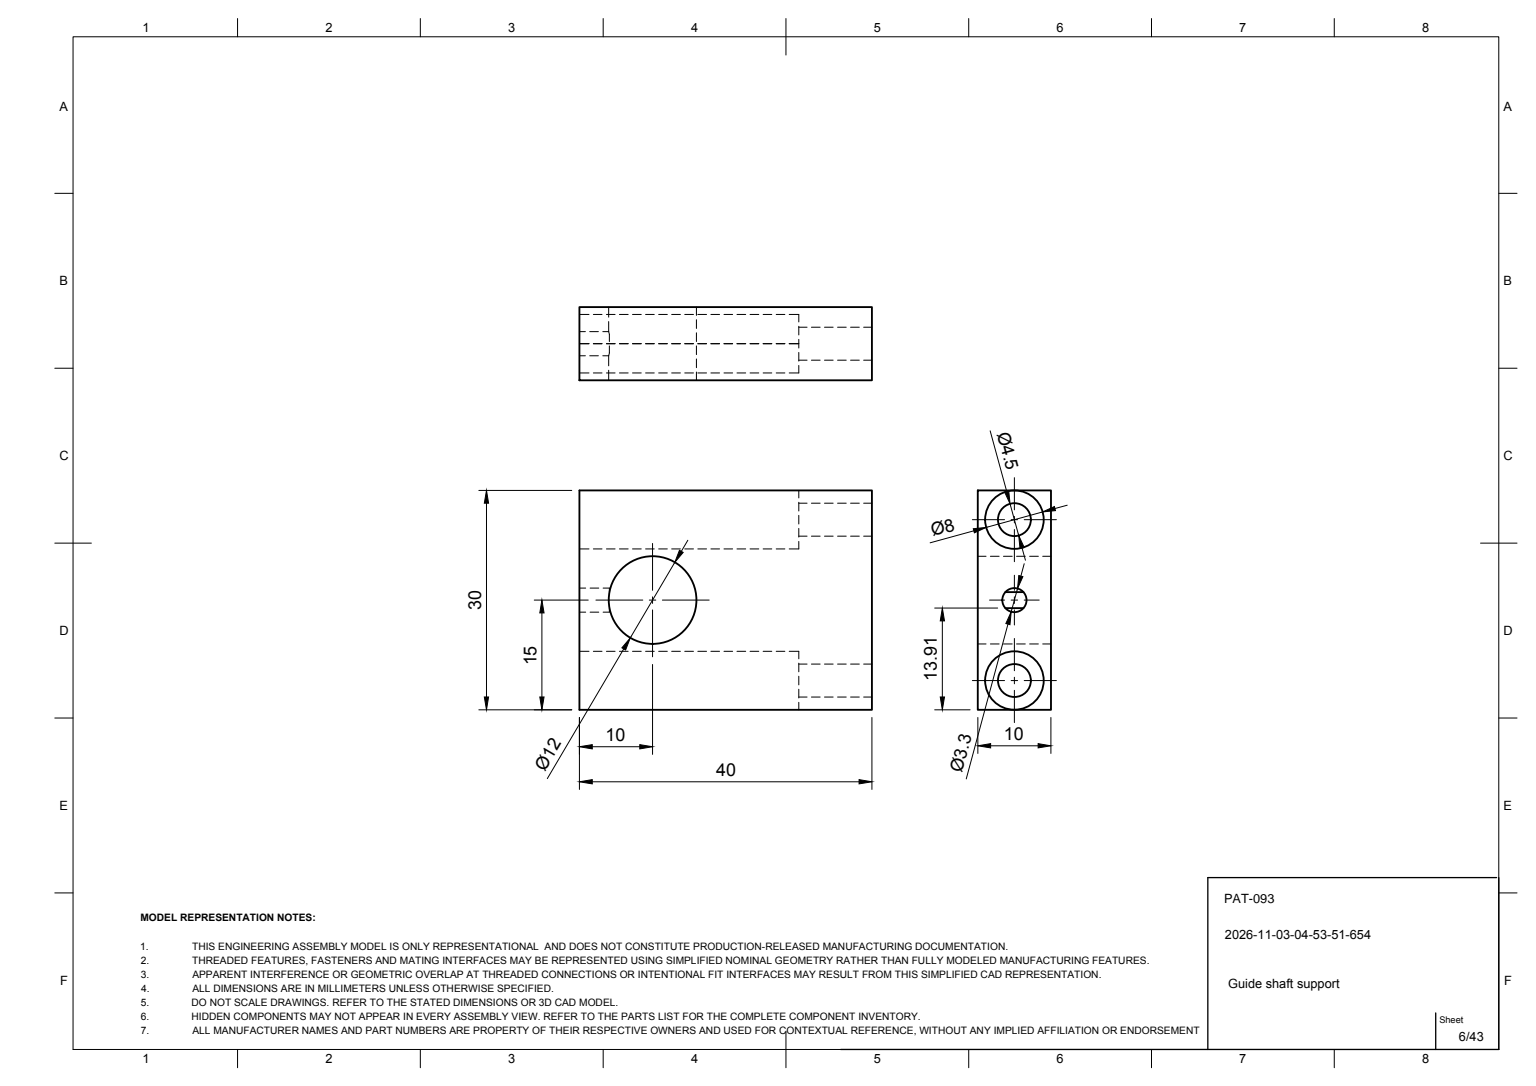
ISO-10303-21;
HEADER;
/* Generated by software containing ST-Developer
 * from STEP Tools, Inc. (www.steptools.com) 
 */

FILE_DESCRIPTION(
/* description */ ('Self-centering screw clamp'),
/* implementation_level */ '2;1');

FILE_NAME(
/* name */ 'Guide shaft support.step',
/* time_stamp */ '2026-10-28T03:25:31-07:00',
/* author */ (''),
/* organization */ (''),
/* preprocessor_version */ 'ST-DEVELOPER v20.2',
/* originating_system */ 'Autodesk Translation Framework v15.17.0.0',
/* authorisation */ '');

FILE_SCHEMA (('AUTOMOTIVE_DESIGN { 1 0 10303 214 3 1 1 }'));
ENDSEC;

DATA;
#10=MECHANICAL_DESIGN_GEOMETRIC_PRESENTATION_REPRESENTATION('',(#627),#16799);
#498=B_SPLINE_CURVE_WITH_KNOTS('',3,(#13857,#13858,#13859,#13860,#13861,
#13862),.UNSPECIFIED.,.F.,.F.,(4,2,4),(0.63543032495593,0.687528937234027,
0.750024497760672),.UNSPECIFIED.);
#499=B_SPLINE_CURVE_WITH_KNOTS('',3,(#13866,#13867,#13868,#13869,#13870,
#13871),.UNSPECIFIED.,.F.,.F.,(4,2,4),(0.250008165920224,0.312503726446869,
0.364602338724965),.UNSPECIFIED.);
#500=B_SPLINE_CURVE_WITH_KNOTS('',3,(#13872,#13873,#13874,#13875,#13876,
#13877),.UNSPECIFIED.,.F.,.F.,(4,2,4),(0.135413993115483,0.187512605393579,
0.250008165920224),.UNSPECIFIED.);
#501=B_SPLINE_CURVE_WITH_KNOTS('',3,(#13878,#13879,#13880,#13881,#13882,
#13883),.UNSPECIFIED.,.F.,.F.,(4,2,4),(0.750024497760672,0.812520058287317,
0.864618670565412),.UNSPECIFIED.);
#545=SHAPE_REPRESENTATION_RELATIONSHIP('SRR','None',#17018,#586);
#586=ADVANCED_BREP_SHAPE_REPRESENTATION('',(#675),#16756);
#627=STYLED_ITEM('',(#17326),#675);
#675=MANIFOLD_SOLID_BREP('Body1',#9078);
#742=FACE_BOUND('',#1838,.T.);
#743=FACE_BOUND('',#1841,.T.);
#744=FACE_BOUND('',#1843,.T.);
#745=FACE_BOUND('',#1849,.T.);
#746=FACE_BOUND('',#1852,.T.);
#747=FACE_BOUND('',#1854,.T.);
#748=FACE_BOUND('',#1855,.T.);
#1032=PLANE('',#9643);
#1033=PLANE('',#9648);
#1034=PLANE('',#9652);
#1035=PLANE('',#9657);
#1036=PLANE('',#9659);
#1037=PLANE('',#9667);
#1038=PLANE('',#9668);
#1039=PLANE('',#9669);
#1040=PLANE('',#9670);
#1041=PLANE('',#9671);
#1303=FACE_OUTER_BOUND('',#1831,.T.);
#1304=FACE_OUTER_BOUND('',#1832,.T.);
#1305=FACE_OUTER_BOUND('',#1833,.T.);
#1306=FACE_OUTER_BOUND('',#1834,.T.);
#1307=FACE_OUTER_BOUND('',#1835,.T.);
#1308=FACE_OUTER_BOUND('',#1836,.T.);
#1309=FACE_OUTER_BOUND('',#1837,.T.);
#1310=FACE_OUTER_BOUND('',#1839,.T.);
#1311=FACE_OUTER_BOUND('',#1840,.T.);
#1312=FACE_OUTER_BOUND('',#1842,.T.);
#1313=FACE_OUTER_BOUND('',#1844,.T.);
#1314=FACE_OUTER_BOUND('',#1845,.T.);
#1315=FACE_OUTER_BOUND('',#1846,.T.);
#1316=FACE_OUTER_BOUND('',#1847,.T.);
#1317=FACE_OUTER_BOUND('',#1848,.T.);
#1318=FACE_OUTER_BOUND('',#1850,.T.);
#1319=FACE_OUTER_BOUND('',#1851,.T.);
#1320=FACE_OUTER_BOUND('',#1853,.T.);
#1831=EDGE_LOOP('',(#6247,#6248,#6249,#6250));
#1832=EDGE_LOOP('',(#6251,#6252,#6253,#6254));
#1833=EDGE_LOOP('',(#6255,#6256));
#1834=EDGE_LOOP('',(#6257,#6258,#6259,#6260,#6261,#6262,#6263,#6264,#6265));
#1835=EDGE_LOOP('',(#6266,#6267));
#1836=EDGE_LOOP('',(#6268,#6269,#6270,#6271));
#1837=EDGE_LOOP('',(#6272,#6273));
#1838=EDGE_LOOP('',(#6274));
#1839=EDGE_LOOP('',(#6275,#6276,#6277,#6278));
#1840=EDGE_LOOP('',(#6279,#6280));
#1841=EDGE_LOOP('',(#6281));
#1842=EDGE_LOOP('',(#6282,#6283,#6284,#6285,#6286,#6287,#6288,#6289,#6290,
#6291));
#1843=EDGE_LOOP('',(#6292));
#1844=EDGE_LOOP('',(#6293,#6294,#6295,#6296));
#1845=EDGE_LOOP('',(#6297,#6298,#6299,#6300));
#1846=EDGE_LOOP('',(#6301,#6302,#6303,#6304,#6305,#6306,#6307,#6308,#6309,
#6310,#6311,#6312));
#1847=EDGE_LOOP('',(#6313,#6314,#6315,#6316,#6317,#6318,#6319));
#1848=EDGE_LOOP('',(#6320,#6321,#6322,#6323));
#1849=EDGE_LOOP('',(#6324));
#1850=EDGE_LOOP('',(#6325,#6326,#6327,#6328,#6329,#6330,#6331));
#1851=EDGE_LOOP('',(#6332,#6333,#6334,#6335));
#1852=EDGE_LOOP('',(#6336));
#1853=EDGE_LOOP('',(#6337,#6338,#6339,#6340));
#1854=EDGE_LOOP('',(#6341));
#1855=EDGE_LOOP('',(#6342));
#2625=LINE('',#13834,#3198);
#2626=LINE('',#13838,#3199);
#2627=LINE('',#13843,#3200);
#2628=LINE('',#13847,#3201);
#2629=LINE('',#13852,#3202);
#2630=LINE('',#13885,#3203);
#2631=LINE('',#13888,#3204);
#2632=LINE('',#13891,#3205);
#2633=LINE('',#13898,#3206);
#2634=LINE('',#13906,#3207);
#2635=LINE('',#13907,#3208);
#2636=LINE('',#13909,#3209);
#2637=LINE('',#13911,#3210);
#2638=LINE('',#13912,#3211);
#2639=LINE('',#13913,#3212);
#2640=LINE('',#13917,#3213);
#2641=LINE('',#13921,#3214);
#2642=LINE('',#13925,#3215);
#2643=LINE('',#13927,#3216);
#2644=LINE('',#13932,#3217);
#2645=LINE('',#13933,#3218);
#2646=LINE('',#13934,#3219);
#2647=LINE('',#13937,#3220);
#2648=LINE('',#13938,#3221);
#2649=LINE('',#13941,#3222);
#2650=LINE('',#13942,#3223);
#2651=LINE('',#13944,#3224);
#3198=VECTOR('',#10922,0.4);
#3199=VECTOR('',#10925,1.);
#3200=VECTOR('',#10930,0.4);
#3201=VECTOR('',#10933,1.);
#3202=VECTOR('',#10938,1.);
#3203=VECTOR('',#10945,0.164999999999999);
#3204=VECTOR('',#10950,1.);
#3205=VECTOR('',#10955,1.);
#3206=VECTOR('',#10966,1.);
#3207=VECTOR('',#10975,1.);
#3208=VECTOR('',#10976,1.);
#3209=VECTOR('',#10977,1.);
#3210=VECTOR('',#10978,1.);
#3211=VECTOR('',#10979,1.);
#3212=VECTOR('',#10980,1.);
#3213=VECTOR('',#10985,0.225);
#3214=VECTOR('',#10990,0.225);
#3215=VECTOR('',#10995,0.6);
#3216=VECTOR('',#10996,0.6);
#3217=VECTOR('',#11001,1.);
#3218=VECTOR('',#11002,1.);
#3219=VECTOR('',#11003,1.);
#3220=VECTOR('',#11006,1.);
#3221=VECTOR('',#11007,1.);
#3222=VECTOR('',#11010,1.);
#3223=VECTOR('',#11011,1.);
#3224=VECTOR('',#11014,1.);
#3747=CIRCLE('',#9638,0.4);
#3748=CIRCLE('',#9639,0.4);
#3749=CIRCLE('',#9641,0.4);
#3750=CIRCLE('',#9642,0.4);
#3751=CIRCLE('',#9644,0.164999999999999);
#3752=CIRCLE('',#9646,0.164999999999999);
#3753=CIRCLE('',#9647,0.164999999999999);
#3754=CIRCLE('',#9650,0.4);
#3755=CIRCLE('',#9651,0.4);
#3756=CIRCLE('',#9653,0.225);
#3757=CIRCLE('',#9655,0.4);
#3758=CIRCLE('',#9656,0.4);
#3759=CIRCLE('',#9658,0.225);
#3760=CIRCLE('',#9661,0.225);
#3761=CIRCLE('',#9663,0.225);
#3762=CIRCLE('',#9665,0.6);
#3763=CIRCLE('',#9666,0.6);
#4281=VERTEX_POINT('',#13832);
#4282=VERTEX_POINT('',#13833);
#4283=VERTEX_POINT('',#13835);
#4284=VERTEX_POINT('',#13837);
#4285=VERTEX_POINT('',#13841);
#4286=VERTEX_POINT('',#13842);
#4287=VERTEX_POINT('',#13844);
#4288=VERTEX_POINT('',#13846);
#4289=VERTEX_POINT('',#13850);
#4290=VERTEX_POINT('',#13851);
#4291=VERTEX_POINT('',#13855);
#4292=VERTEX_POINT('',#13856);
#4293=VERTEX_POINT('',#13863);
#4294=VERTEX_POINT('',#13865);
#4295=VERTEX_POINT('',#13884);
#4296=VERTEX_POINT('',#13894);
#4297=VERTEX_POINT('',#13901);
#4298=VERTEX_POINT('',#13904);
#4299=VERTEX_POINT('',#13905);
#4300=VERTEX_POINT('',#13908);
#4301=VERTEX_POINT('',#13910);
#4302=VERTEX_POINT('',#13915);
#4303=VERTEX_POINT('',#13919);
#4304=VERTEX_POINT('',#13923);
#4305=VERTEX_POINT('',#13926);
#4306=VERTEX_POINT('',#13930);
#4307=VERTEX_POINT('',#13931);
#4308=VERTEX_POINT('',#13936);
#4309=VERTEX_POINT('',#13940);
#5048=EDGE_CURVE('',#4281,#4282,#2625,.T.);
#5049=EDGE_CURVE('',#4283,#4281,#3747,.T.);
#5050=EDGE_CURVE('',#4283,#4284,#2626,.T.);
#5051=EDGE_CURVE('',#4282,#4284,#3748,.T.);
#5052=EDGE_CURVE('',#4285,#4286,#2627,.T.);
#5053=EDGE_CURVE('',#4287,#4285,#3749,.T.);
#5054=EDGE_CURVE('',#4287,#4288,#2628,.T.);
#5055=EDGE_CURVE('',#4286,#4288,#3750,.T.);
#5056=EDGE_CURVE('',#4289,#4290,#2629,.T.);
#5057=EDGE_CURVE('',#4289,#4290,#3751,.T.);
#5058=EDGE_CURVE('',#4291,#4292,#498,.T.);
#5059=EDGE_CURVE('',#4293,#4291,#3752,.T.);
#5060=EDGE_CURVE('',#4294,#4293,#499,.T.);
#5061=EDGE_CURVE('',#4290,#4294,#500,.T.);
#5062=EDGE_CURVE('',#4292,#4289,#501,.T.);
#5063=EDGE_CURVE('',#4292,#4295,#2630,.T.);
#5064=EDGE_CURVE('',#4295,#4295,#3753,.T.);
#5065=EDGE_CURVE('',#4293,#4291,#2631,.T.);
#5066=EDGE_CURVE('',#4288,#4286,#3754,.T.);
#5067=EDGE_CURVE('',#4287,#4288,#2632,.T.);
#5068=EDGE_CURVE('',#4285,#4287,#3755,.T.);
#5069=EDGE_CURVE('',#4296,#4296,#3756,.T.);
#5070=EDGE_CURVE('',#4284,#4282,#3757,.T.);
#5071=EDGE_CURVE('',#4283,#4284,#2633,.T.);
#5072=EDGE_CURVE('',#4281,#4283,#3758,.T.);
#5073=EDGE_CURVE('',#4297,#4297,#3759,.T.);
#5074=EDGE_CURVE('',#4298,#4299,#2634,.T.);
#5075=EDGE_CURVE('',#4299,#4288,#2635,.T.);
#5076=EDGE_CURVE('',#4288,#4300,#2636,.T.);
#5077=EDGE_CURVE('',#4300,#4301,#2637,.T.);
#5078=EDGE_CURVE('',#4301,#4284,#2638,.T.);
#5079=EDGE_CURVE('',#4284,#4298,#2639,.T.);
#5080=EDGE_CURVE('',#4302,#4302,#3760,.T.);
#5081=EDGE_CURVE('',#4302,#4296,#2640,.T.);
#5082=EDGE_CURVE('',#4303,#4303,#3761,.T.);
#5083=EDGE_CURVE('',#4303,#4297,#2641,.T.);
#5084=EDGE_CURVE('',#4304,#4304,#3762,.T.);
#5085=EDGE_CURVE('',#4304,#4292,#2642,.T.);
#5086=EDGE_CURVE('',#4294,#4305,#2643,.T.);
#5087=EDGE_CURVE('',#4305,#4305,#3763,.T.);
#5088=EDGE_CURVE('',#4306,#4307,#2644,.T.);
#5089=EDGE_CURVE('',#4307,#4298,#2645,.T.);
#5090=EDGE_CURVE('',#4306,#4301,#2646,.T.);
#5091=EDGE_CURVE('',#4308,#4306,#2647,.T.);
#5092=EDGE_CURVE('',#4308,#4300,#2648,.T.);
#5093=EDGE_CURVE('',#4309,#4308,#2649,.T.);
#5094=EDGE_CURVE('',#4309,#4299,#2650,.T.);
#5095=EDGE_CURVE('',#4307,#4309,#2651,.T.);
#6247=ORIENTED_EDGE('',*,*,#5048,.F.);
#6248=ORIENTED_EDGE('',*,*,#5049,.F.);
#6249=ORIENTED_EDGE('',*,*,#5050,.T.);
#6250=ORIENTED_EDGE('',*,*,#5051,.F.);
#6251=ORIENTED_EDGE('',*,*,#5052,.F.);
#6252=ORIENTED_EDGE('',*,*,#5053,.F.);
#6253=ORIENTED_EDGE('',*,*,#5054,.T.);
#6254=ORIENTED_EDGE('',*,*,#5055,.F.);
#6255=ORIENTED_EDGE('',*,*,#5056,.F.);
#6256=ORIENTED_EDGE('',*,*,#5057,.T.);
#6257=ORIENTED_EDGE('',*,*,#5058,.F.);
#6258=ORIENTED_EDGE('',*,*,#5059,.F.);
#6259=ORIENTED_EDGE('',*,*,#5060,.F.);
#6260=ORIENTED_EDGE('',*,*,#5061,.F.);
#6261=ORIENTED_EDGE('',*,*,#5057,.F.);
#6262=ORIENTED_EDGE('',*,*,#5062,.F.);
#6263=ORIENTED_EDGE('',*,*,#5063,.T.);
#6264=ORIENTED_EDGE('',*,*,#5064,.F.);
#6265=ORIENTED_EDGE('',*,*,#5063,.F.);
#6266=ORIENTED_EDGE('',*,*,#5065,.F.);
#6267=ORIENTED_EDGE('',*,*,#5059,.T.);
#6268=ORIENTED_EDGE('',*,*,#5052,.T.);
#6269=ORIENTED_EDGE('',*,*,#5066,.F.);
#6270=ORIENTED_EDGE('',*,*,#5067,.F.);
#6271=ORIENTED_EDGE('',*,*,#5068,.F.);
#6272=ORIENTED_EDGE('',*,*,#5053,.T.);
#6273=ORIENTED_EDGE('',*,*,#5068,.T.);
#6274=ORIENTED_EDGE('',*,*,#5069,.F.);
#6275=ORIENTED_EDGE('',*,*,#5048,.T.);
#6276=ORIENTED_EDGE('',*,*,#5070,.F.);
#6277=ORIENTED_EDGE('',*,*,#5071,.F.);
#6278=ORIENTED_EDGE('',*,*,#5072,.F.);
#6279=ORIENTED_EDGE('',*,*,#5049,.T.);
#6280=ORIENTED_EDGE('',*,*,#5072,.T.);
#6281=ORIENTED_EDGE('',*,*,#5073,.F.);
#6282=ORIENTED_EDGE('',*,*,#5074,.T.);
#6283=ORIENTED_EDGE('',*,*,#5075,.T.);
#6284=ORIENTED_EDGE('',*,*,#5066,.T.);
#6285=ORIENTED_EDGE('',*,*,#5055,.T.);
#6286=ORIENTED_EDGE('',*,*,#5076,.T.);
#6287=ORIENTED_EDGE('',*,*,#5077,.T.);
#6288=ORIENTED_EDGE('',*,*,#5078,.T.);
#6289=ORIENTED_EDGE('',*,*,#5070,.T.);
#6290=ORIENTED_EDGE('',*,*,#5051,.T.);
#6291=ORIENTED_EDGE('',*,*,#5079,.T.);
#6292=ORIENTED_EDGE('',*,*,#5064,.T.);
#6293=ORIENTED_EDGE('',*,*,#5080,.F.);
#6294=ORIENTED_EDGE('',*,*,#5081,.T.);
#6295=ORIENTED_EDGE('',*,*,#5069,.T.);
#6296=ORIENTED_EDGE('',*,*,#5081,.F.);
#6297=ORIENTED_EDGE('',*,*,#5082,.F.);
#6298=ORIENTED_EDGE('',*,*,#5083,.T.);
#6299=ORIENTED_EDGE('',*,*,#5073,.T.);
#6300=ORIENTED_EDGE('',*,*,#5083,.F.);
#6301=ORIENTED_EDGE('',*,*,#5084,.F.);
#6302=ORIENTED_EDGE('',*,*,#5085,.T.);
#6303=ORIENTED_EDGE('',*,*,#5062,.T.);
#6304=ORIENTED_EDGE('',*,*,#5056,.T.);
#6305=ORIENTED_EDGE('',*,*,#5061,.T.);
#6306=ORIENTED_EDGE('',*,*,#5086,.T.);
#6307=ORIENTED_EDGE('',*,*,#5087,.F.);
#6308=ORIENTED_EDGE('',*,*,#5086,.F.);
#6309=ORIENTED_EDGE('',*,*,#5060,.T.);
#6310=ORIENTED_EDGE('',*,*,#5065,.T.);
#6311=ORIENTED_EDGE('',*,*,#5058,.T.);
#6312=ORIENTED_EDGE('',*,*,#5085,.F.);
#6313=ORIENTED_EDGE('',*,*,#5088,.T.);
#6314=ORIENTED_EDGE('',*,*,#5089,.T.);
#6315=ORIENTED_EDGE('',*,*,#5079,.F.);
#6316=ORIENTED_EDGE('',*,*,#5050,.F.);
#6317=ORIENTED_EDGE('',*,*,#5071,.T.);
#6318=ORIENTED_EDGE('',*,*,#5078,.F.);
#6319=ORIENTED_EDGE('',*,*,#5090,.F.);
#6320=ORIENTED_EDGE('',*,*,#5091,.T.);
#6321=ORIENTED_EDGE('',*,*,#5090,.T.);
#6322=ORIENTED_EDGE('',*,*,#5077,.F.);
#6323=ORIENTED_EDGE('',*,*,#5092,.F.);
#6324=ORIENTED_EDGE('',*,*,#5087,.T.);
#6325=ORIENTED_EDGE('',*,*,#5093,.T.);
#6326=ORIENTED_EDGE('',*,*,#5092,.T.);
#6327=ORIENTED_EDGE('',*,*,#5076,.F.);
#6328=ORIENTED_EDGE('',*,*,#5054,.F.);
#6329=ORIENTED_EDGE('',*,*,#5067,.T.);
#6330=ORIENTED_EDGE('',*,*,#5075,.F.);
#6331=ORIENTED_EDGE('',*,*,#5094,.F.);
#6332=ORIENTED_EDGE('',*,*,#5095,.T.);
#6333=ORIENTED_EDGE('',*,*,#5094,.T.);
#6334=ORIENTED_EDGE('',*,*,#5074,.F.);
#6335=ORIENTED_EDGE('',*,*,#5089,.F.);
#6336=ORIENTED_EDGE('',*,*,#5084,.T.);
#6337=ORIENTED_EDGE('',*,*,#5095,.F.);
#6338=ORIENTED_EDGE('',*,*,#5088,.F.);
#6339=ORIENTED_EDGE('',*,*,#5091,.F.);
#6340=ORIENTED_EDGE('',*,*,#5093,.F.);
#6341=ORIENTED_EDGE('',*,*,#5080,.T.);
#6342=ORIENTED_EDGE('',*,*,#5082,.T.);
#8369=CYLINDRICAL_SURFACE('',#9637,0.4);
#8370=CYLINDRICAL_SURFACE('',#9640,0.4);
#8371=CYLINDRICAL_SURFACE('',#9645,0.164999999999999);
#8372=CYLINDRICAL_SURFACE('',#9649,0.4);
#8373=CYLINDRICAL_SURFACE('',#9654,0.4);
#8374=CYLINDRICAL_SURFACE('',#9660,0.225);
#8375=CYLINDRICAL_SURFACE('',#9662,0.225);
#8376=CYLINDRICAL_SURFACE('',#9664,0.6);
#8601=ADVANCED_FACE('',(#1303),#8369,.F.);
#8602=ADVANCED_FACE('',(#1304),#8370,.F.);
#8603=ADVANCED_FACE('',(#1305),#1032,.T.);
#8604=ADVANCED_FACE('',(#1306),#8371,.F.);
#8605=ADVANCED_FACE('',(#1307),#1033,.T.);
#8606=ADVANCED_FACE('',(#1308),#8372,.F.);
#8607=ADVANCED_FACE('',(#1309,#742),#1034,.T.);
#8608=ADVANCED_FACE('',(#1310),#8373,.F.);
#8609=ADVANCED_FACE('',(#1311,#743),#1035,.T.);
#8610=ADVANCED_FACE('',(#1312,#744),#1036,.T.);
#8611=ADVANCED_FACE('',(#1313),#8374,.F.);
#8612=ADVANCED_FACE('',(#1314),#8375,.F.);
#8613=ADVANCED_FACE('',(#1315),#8376,.F.);
#8614=ADVANCED_FACE('',(#1316),#1037,.T.);
#8615=ADVANCED_FACE('',(#1317,#745),#1038,.T.);
#8616=ADVANCED_FACE('',(#1318),#1039,.T.);
#8617=ADVANCED_FACE('',(#1319,#746),#1040,.T.);
#8618=ADVANCED_FACE('',(#1320,#747,#748),#1041,.F.);
#9078=CLOSED_SHELL('',(#8601,#8602,#8603,#8604,#8605,#8606,#8607,#8608,
#8609,#8610,#8611,#8612,#8613,#8614,#8615,#8616,#8617,#8618));
#9636=AXIS2_PLACEMENT_3D('',#13830,#10918,#10919);
#9637=AXIS2_PLACEMENT_3D('',#13831,#10920,#10921);
#9638=AXIS2_PLACEMENT_3D('',#13836,#10923,#10924);
#9639=AXIS2_PLACEMENT_3D('',#13839,#10926,#10927);
#9640=AXIS2_PLACEMENT_3D('',#13840,#10928,#10929);
#9641=AXIS2_PLACEMENT_3D('',#13845,#10931,#10932);
#9642=AXIS2_PLACEMENT_3D('',#13848,#10934,#10935);
#9643=AXIS2_PLACEMENT_3D('',#13849,#10936,#10937);
#9644=AXIS2_PLACEMENT_3D('',#13853,#10939,#10940);
#9645=AXIS2_PLACEMENT_3D('',#13854,#10941,#10942);
#9646=AXIS2_PLACEMENT_3D('',#13864,#10943,#10944);
#9647=AXIS2_PLACEMENT_3D('',#13886,#10946,#10947);
#9648=AXIS2_PLACEMENT_3D('',#13887,#10948,#10949);
#9649=AXIS2_PLACEMENT_3D('',#13889,#10951,#10952);
#9650=AXIS2_PLACEMENT_3D('',#13890,#10953,#10954);
#9651=AXIS2_PLACEMENT_3D('',#13892,#10956,#10957);
#9652=AXIS2_PLACEMENT_3D('',#13893,#10958,#10959);
#9653=AXIS2_PLACEMENT_3D('',#13895,#10960,#10961);
#9654=AXIS2_PLACEMENT_3D('',#13896,#10962,#10963);
#9655=AXIS2_PLACEMENT_3D('',#13897,#10964,#10965);
#9656=AXIS2_PLACEMENT_3D('',#13899,#10967,#10968);
#9657=AXIS2_PLACEMENT_3D('',#13900,#10969,#10970);
#9658=AXIS2_PLACEMENT_3D('',#13902,#10971,#10972);
#9659=AXIS2_PLACEMENT_3D('',#13903,#10973,#10974);
#9660=AXIS2_PLACEMENT_3D('',#13914,#10981,#10982);
#9661=AXIS2_PLACEMENT_3D('',#13916,#10983,#10984);
#9662=AXIS2_PLACEMENT_3D('',#13918,#10986,#10987);
#9663=AXIS2_PLACEMENT_3D('',#13920,#10988,#10989);
#9664=AXIS2_PLACEMENT_3D('',#13922,#10991,#10992);
#9665=AXIS2_PLACEMENT_3D('',#13924,#10993,#10994);
#9666=AXIS2_PLACEMENT_3D('',#13928,#10997,#10998);
#9667=AXIS2_PLACEMENT_3D('',#13929,#10999,#11000);
#9668=AXIS2_PLACEMENT_3D('',#13935,#11004,#11005);
#9669=AXIS2_PLACEMENT_3D('',#13939,#11008,#11009);
#9670=AXIS2_PLACEMENT_3D('',#13943,#11012,#11013);
#9671=AXIS2_PLACEMENT_3D('',#13945,#11015,#11016);
#10918=DIRECTION('axis',(0.,0.,1.));
#10919=DIRECTION('refdir',(1.,0.,0.));
#10920=DIRECTION('center_axis',(0.,0.,1.));
#10921=DIRECTION('ref_axis',(1.,0.,0.));
#10922=DIRECTION('',(0.,0.,1.));
#10923=DIRECTION('center_axis',(0.,0.,1.));
#10924=DIRECTION('ref_axis',(1.,0.,0.));
#10925=DIRECTION('',(0.,0.,1.));
#10926=DIRECTION('center_axis',(0.,0.,-1.));
#10927=DIRECTION('ref_axis',(1.,0.,0.));
#10928=DIRECTION('center_axis',(0.,0.,1.));
#10929=DIRECTION('ref_axis',(1.,0.,0.));
#10930=DIRECTION('',(0.,0.,1.));
#10931=DIRECTION('center_axis',(0.,0.,1.));
#10932=DIRECTION('ref_axis',(1.,0.,0.));
#10933=DIRECTION('',(0.,0.,1.));
#10934=DIRECTION('center_axis',(0.,0.,-1.));
#10935=DIRECTION('ref_axis',(1.,0.,0.));
#10936=DIRECTION('center_axis',(0.,0.,1.));
#10937=DIRECTION('ref_axis',(1.,0.,0.));
#10938=DIRECTION('',(1.,0.,0.));
#10939=DIRECTION('center_axis',(0.,0.,1.));
#10940=DIRECTION('ref_axis',(1.,0.,0.));
#10941=DIRECTION('center_axis',(0.,0.,1.));
#10942=DIRECTION('ref_axis',(1.,0.,0.));
#10943=DIRECTION('center_axis',(0.,0.,1.));
#10944=DIRECTION('ref_axis',(1.,0.,0.));
#10945=DIRECTION('',(0.,0.,1.));
#10946=DIRECTION('center_axis',(0.,0.,-1.));
#10947=DIRECTION('ref_axis',(1.,0.,0.));
#10948=DIRECTION('center_axis',(0.,0.,1.));
#10949=DIRECTION('ref_axis',(1.,0.,0.));
#10950=DIRECTION('',(-1.,0.,0.));
#10951=DIRECTION('center_axis',(0.,0.,1.));
#10952=DIRECTION('ref_axis',(1.,0.,0.));
#10953=DIRECTION('center_axis',(0.,0.,-1.));
#10954=DIRECTION('ref_axis',(1.,0.,0.));
#10955=DIRECTION('',(0.,0.,1.));
#10956=DIRECTION('center_axis',(0.,0.,1.));
#10957=DIRECTION('ref_axis',(1.,0.,0.));
#10958=DIRECTION('center_axis',(0.,0.,1.));
#10959=DIRECTION('ref_axis',(1.,0.,0.));
#10960=DIRECTION('center_axis',(0.,0.,1.));
#10961=DIRECTION('ref_axis',(1.,0.,0.));
#10962=DIRECTION('center_axis',(0.,0.,1.));
#10963=DIRECTION('ref_axis',(1.,0.,0.));
#10964=DIRECTION('center_axis',(0.,0.,-1.));
#10965=DIRECTION('ref_axis',(1.,0.,0.));
#10966=DIRECTION('',(0.,0.,1.));
#10967=DIRECTION('center_axis',(0.,0.,1.));
#10968=DIRECTION('ref_axis',(1.,0.,0.));
#10969=DIRECTION('center_axis',(0.,0.,1.));
#10970=DIRECTION('ref_axis',(1.,0.,0.));
#10971=DIRECTION('center_axis',(0.,0.,1.));
#10972=DIRECTION('ref_axis',(1.,0.,0.));
#10973=DIRECTION('center_axis',(0.,0.,1.));
#10974=DIRECTION('ref_axis',(1.,0.,0.));
#10975=DIRECTION('',(0.,-1.,0.));
#10976=DIRECTION('',(1.,0.,0.));
#10977=DIRECTION('',(1.,0.,0.));
#10978=DIRECTION('',(0.,1.,0.));
#10979=DIRECTION('',(-1.,0.,0.));
#10980=DIRECTION('',(-1.,0.,0.));
#10981=DIRECTION('center_axis',(0.,0.,1.));
#10982=DIRECTION('ref_axis',(1.,0.,0.));
#10983=DIRECTION('center_axis',(0.,0.,1.));
#10984=DIRECTION('ref_axis',(1.,0.,0.));
#10985=DIRECTION('',(0.,0.,1.));
#10986=DIRECTION('center_axis',(0.,0.,1.));
#10987=DIRECTION('ref_axis',(1.,0.,0.));
#10988=DIRECTION('center_axis',(0.,0.,1.));
#10989=DIRECTION('ref_axis',(1.,0.,0.));
#10990=DIRECTION('',(0.,0.,1.));
#10991=DIRECTION('center_axis',(1.,0.,0.));
#10992=DIRECTION('ref_axis',(0.,0.,-1.));
#10993=DIRECTION('center_axis',(1.,0.,0.));
#10994=DIRECTION('ref_axis',(0.,0.,-1.));
#10995=DIRECTION('',(1.,0.,0.));
#10996=DIRECTION('',(1.,0.,0.));
#10997=DIRECTION('center_axis',(-1.,0.,0.));
#10998=DIRECTION('ref_axis',(0.,0.,-1.));
#10999=DIRECTION('center_axis',(0.,1.,0.));
#11000=DIRECTION('ref_axis',(-1.,0.,0.));
#11001=DIRECTION('',(-1.,0.,0.));
#11002=DIRECTION('',(0.,0.,1.));
#11003=DIRECTION('',(0.,0.,1.));
#11004=DIRECTION('center_axis',(1.,0.,0.));
#11005=DIRECTION('ref_axis',(0.,1.,0.));
#11006=DIRECTION('',(0.,1.,0.));
#11007=DIRECTION('',(0.,0.,1.));
#11008=DIRECTION('center_axis',(0.,-1.,0.));
#11009=DIRECTION('ref_axis',(1.,0.,0.));
#11010=DIRECTION('',(1.,0.,0.));
#11011=DIRECTION('',(0.,0.,1.));
#11012=DIRECTION('center_axis',(-1.,0.,0.));
#11013=DIRECTION('ref_axis',(0.,-1.,0.));
#11014=DIRECTION('',(0.,-1.,0.));
#11015=DIRECTION('center_axis',(0.,0.,1.));
#11016=DIRECTION('ref_axis',(1.,0.,0.));
#13830=CARTESIAN_POINT('',(0.,0.,0.));
#13831=CARTESIAN_POINT('Origin',(-13.5,-1.9,2.));
#13832=CARTESIAN_POINT('',(-13.9,-1.9,2.));
#13833=CARTESIAN_POINT('',(-13.9,-1.9,5.));
#13834=CARTESIAN_POINT('',(-13.9,-1.9,2.));
#13835=CARTESIAN_POINT('',(-13.5,-1.5,2.));
#13836=CARTESIAN_POINT('Origin',(-13.5,-1.9,2.));
#13837=CARTESIAN_POINT('',(-13.5,-1.5,5.));
#13838=CARTESIAN_POINT('',(-13.5,-1.5,2.));
#13839=CARTESIAN_POINT('Origin',(-13.5,-1.9,5.));
#13840=CARTESIAN_POINT('Origin',(-13.5,-4.1,2.));
#13841=CARTESIAN_POINT('',(-13.9,-4.1,2.));
#13842=CARTESIAN_POINT('',(-13.9,-4.1,5.));
#13843=CARTESIAN_POINT('',(-13.9,-4.1,2.));
#13844=CARTESIAN_POINT('',(-13.5,-4.5,2.));
#13845=CARTESIAN_POINT('Origin',(-13.5,-4.1,2.));
#13846=CARTESIAN_POINT('',(-13.5,-4.5,5.));
#13847=CARTESIAN_POINT('',(-13.5,-4.5,2.));
#13848=CARTESIAN_POINT('Origin',(-13.5,-4.1,5.));
#13849=CARTESIAN_POINT('Origin',(-13.5,-3.,4.59));
#13850=CARTESIAN_POINT('',(-13.6237941840314,-3.10908712114636,4.59));
#13851=CARTESIAN_POINT('',(-13.3762058159686,-3.10908712114636,4.59));
#13852=CARTESIAN_POINT('',(-14.1,-3.10908712114636,4.59));
#13853=CARTESIAN_POINT('Origin',(-13.5,-3.,4.59));
#13854=CARTESIAN_POINT('Origin',(-13.5,-3.,4.59));
#13855=CARTESIAN_POINT('',(-13.6237941840314,-2.89091287885364,4.59));
#13856=CARTESIAN_POINT('',(-13.665,-3.,4.6));
#13857=CARTESIAN_POINT('Ctrl Pts',(-13.6237941840314,-2.89091287885364,
4.59));
#13858=CARTESIAN_POINT('Ctrl Pts',(-13.6353991351895,-2.90408240284739,
4.59243495840567));
#13859=CARTESIAN_POINT('Ctrl Pts',(-13.6453456436582,-2.91977655056228,
4.59485638705045));
#13860=CARTESIAN_POINT('Ctrl Pts',(-13.660814864634,-2.95701983403981,4.59880705606552));
#13861=CARTESIAN_POINT('Ctrl Pts',(-13.665,-2.97916814649112,4.6));
#13862=CARTESIAN_POINT('Ctrl Pts',(-13.665,-3.,4.6));
#13863=CARTESIAN_POINT('',(-13.3762058159686,-2.89091287885364,4.59));
#13864=CARTESIAN_POINT('Origin',(-13.5,-3.,4.59));
#13865=CARTESIAN_POINT('',(-13.335,-3.,4.6));
#13866=CARTESIAN_POINT('Ctrl Pts',(-13.335,-3.,4.6));
#13867=CARTESIAN_POINT('Ctrl Pts',(-13.335,-2.97916814649112,4.6));
#13868=CARTESIAN_POINT('Ctrl Pts',(-13.339185135366,-2.95701983403981,4.59880705606552));
#13869=CARTESIAN_POINT('Ctrl Pts',(-13.3546543563418,-2.91977655056228,
4.59485638705045));
#13870=CARTESIAN_POINT('Ctrl Pts',(-13.3646008648105,-2.90408240284739,
4.59243495840567));
#13871=CARTESIAN_POINT('Ctrl Pts',(-13.3762058159686,-2.89091287885364,
4.59));
#13872=CARTESIAN_POINT('Ctrl Pts',(-13.3762058159686,-3.10908712114636,
4.59));
#13873=CARTESIAN_POINT('Ctrl Pts',(-13.3646008648105,-3.09591759715261,
4.59243495840567));
#13874=CARTESIAN_POINT('Ctrl Pts',(-13.3546543563418,-3.08022344943772,
4.59485638705045));
#13875=CARTESIAN_POINT('Ctrl Pts',(-13.339185135366,-3.04298016596019,4.59880705606552));
#13876=CARTESIAN_POINT('Ctrl Pts',(-13.335,-3.02083185350888,4.6));
#13877=CARTESIAN_POINT('Ctrl Pts',(-13.335,-3.,4.6));
#13878=CARTESIAN_POINT('Ctrl Pts',(-13.665,-3.,4.6));
#13879=CARTESIAN_POINT('Ctrl Pts',(-13.665,-3.02083185350888,4.6));
#13880=CARTESIAN_POINT('Ctrl Pts',(-13.660814864634,-3.04298016596019,4.59880705606552));
#13881=CARTESIAN_POINT('Ctrl Pts',(-13.6453456436582,-3.08022344943772,
4.59485638705045));
#13882=CARTESIAN_POINT('Ctrl Pts',(-13.6353991351895,-3.09591759715261,
4.59243495840567));
#13883=CARTESIAN_POINT('Ctrl Pts',(-13.6237941840314,-3.10908712114636,
4.59));
#13884=CARTESIAN_POINT('',(-13.665,-3.,5.));
#13885=CARTESIAN_POINT('',(-13.665,-3.,4.59));
#13886=CARTESIAN_POINT('Origin',(-13.5,-3.,5.));
#13887=CARTESIAN_POINT('Origin',(-13.5,-3.,4.59));
#13888=CARTESIAN_POINT('',(-14.1,-2.89091287885364,4.59));
#13889=CARTESIAN_POINT('Origin',(-13.5,-4.1,2.));
#13890=CARTESIAN_POINT('Origin',(-13.5,-4.1,5.));
#13891=CARTESIAN_POINT('',(-13.5,-4.5,2.));
#13892=CARTESIAN_POINT('Origin',(-13.5,-4.1,2.));
#13893=CARTESIAN_POINT('Origin',(-13.5,-4.1,2.));
#13894=CARTESIAN_POINT('',(-13.725,-4.1,2.));
#13895=CARTESIAN_POINT('Origin',(-13.5,-4.1,2.));
#13896=CARTESIAN_POINT('Origin',(-13.5,-1.9,2.));
#13897=CARTESIAN_POINT('Origin',(-13.5,-1.9,5.));
#13898=CARTESIAN_POINT('',(-13.5,-1.5,2.));
#13899=CARTESIAN_POINT('Origin',(-13.5,-1.9,2.));
#13900=CARTESIAN_POINT('Origin',(-13.5,-1.9,2.));
#13901=CARTESIAN_POINT('',(-13.725,-1.9,2.));
#13902=CARTESIAN_POINT('Origin',(-13.5,-1.9,2.));
#13903=CARTESIAN_POINT('Origin',(-13.5,-3.,5.));
#13904=CARTESIAN_POINT('',(-14.,-1.5,5.));
#13905=CARTESIAN_POINT('',(-14.,-4.5,5.));
#13906=CARTESIAN_POINT('',(-14.,-1.5,5.));
#13907=CARTESIAN_POINT('',(-14.,-4.5,5.));
#13908=CARTESIAN_POINT('',(-13.,-4.5,5.));
#13909=CARTESIAN_POINT('',(-14.,-4.5,5.));
#13910=CARTESIAN_POINT('',(-13.,-1.5,5.));
#13911=CARTESIAN_POINT('',(-13.,-4.5,5.));
#13912=CARTESIAN_POINT('',(-13.,-1.5,5.));
#13913=CARTESIAN_POINT('',(-13.,-1.5,5.));
#13914=CARTESIAN_POINT('Origin',(-13.5,-4.1,0.9));
#13915=CARTESIAN_POINT('',(-13.725,-4.1,1.));
#13916=CARTESIAN_POINT('Origin',(-13.5,-4.1,1.));
#13917=CARTESIAN_POINT('',(-13.725,-4.1,0.9));
#13918=CARTESIAN_POINT('Origin',(-13.5,-1.9,0.9));
#13919=CARTESIAN_POINT('',(-13.725,-1.9,1.));
#13920=CARTESIAN_POINT('Origin',(-13.5,-1.9,1.));
#13921=CARTESIAN_POINT('',(-13.725,-1.9,0.9));
#13922=CARTESIAN_POINT('Origin',(-14.1,-3.,4.));
#13923=CARTESIAN_POINT('',(-14.,-3.,4.6));
#13924=CARTESIAN_POINT('Origin',(-14.,-3.,4.));
#13925=CARTESIAN_POINT('',(-14.1,-3.,4.6));
#13926=CARTESIAN_POINT('',(-13.,-3.,4.6));
#13927=CARTESIAN_POINT('',(-14.1,-3.,4.6));
#13928=CARTESIAN_POINT('Origin',(-13.,-3.,4.));
#13929=CARTESIAN_POINT('Origin',(-13.,-1.5,1.));
#13930=CARTESIAN_POINT('',(-13.,-1.5,1.));
#13931=CARTESIAN_POINT('',(-14.,-1.5,1.));
#13932=CARTESIAN_POINT('',(-13.,-1.5,1.));
#13933=CARTESIAN_POINT('',(-14.,-1.5,1.));
#13934=CARTESIAN_POINT('',(-13.,-1.5,1.));
#13935=CARTESIAN_POINT('Origin',(-13.,-4.5,1.));
#13936=CARTESIAN_POINT('',(-13.,-4.5,1.));
#13937=CARTESIAN_POINT('',(-13.,-4.5,1.));
#13938=CARTESIAN_POINT('',(-13.,-4.5,1.));
#13939=CARTESIAN_POINT('Origin',(-14.,-4.5,1.));
#13940=CARTESIAN_POINT('',(-14.,-4.5,1.));
#13941=CARTESIAN_POINT('',(-14.,-4.5,1.));
#13942=CARTESIAN_POINT('',(-14.,-4.5,1.));
#13943=CARTESIAN_POINT('Origin',(-14.,-1.5,1.));
#13944=CARTESIAN_POINT('',(-14.,-1.5,1.));
#13945=CARTESIAN_POINT('Origin',(-13.5,-3.,1.));
#16707=UNCERTAINTY_MEASURE_WITH_UNIT(LENGTH_MEASURE(0.001),#16800,
'DISTANCE_ACCURACY_VALUE',
'Maximum model space distance between geometric entities at asserted c
onnectivities');
#16750=UNCERTAINTY_MEASURE_WITH_UNIT(LENGTH_MEASURE(0.001),#16800,
'DISTANCE_ACCURACY_VALUE',
'Maximum model space distance between geometric entities at asserted c
onnectivities');
#16756=(
GEOMETRIC_REPRESENTATION_CONTEXT(3)
GLOBAL_UNCERTAINTY_ASSIGNED_CONTEXT((#16707))
GLOBAL_UNIT_ASSIGNED_CONTEXT((#16800,#16802,#16803))
REPRESENTATION_CONTEXT('','3D')
);
#16799=(
GEOMETRIC_REPRESENTATION_CONTEXT(3)
GLOBAL_UNCERTAINTY_ASSIGNED_CONTEXT((#16750))
GLOBAL_UNIT_ASSIGNED_CONTEXT((#16800,#16802,#16803))
REPRESENTATION_CONTEXT('','3D')
);
#16800=(
LENGTH_UNIT()
NAMED_UNIT(*)
SI_UNIT(.CENTI.,.METRE.)
);
#16802=(
NAMED_UNIT(*)
PLANE_ANGLE_UNIT()
SI_UNIT($,.RADIAN.)
);
#16803=(
NAMED_UNIT(*)
SI_UNIT($,.STERADIAN.)
SOLID_ANGLE_UNIT()
);
#16809=SHAPE_DEFINITION_REPRESENTATION(#16857,#17018);
#16857=PRODUCT_DEFINITION_SHAPE('',$,#17067);
#17018=SHAPE_REPRESENTATION('',(#9636),#16756);
#17061=PRODUCT_DEFINITION_CONTEXT('part definition',#17207,'design');
#17067=PRODUCT_DEFINITION('Guide shaft support','Guide shaft support',#17115,
#17061);
#17115=PRODUCT_DEFINITION_FORMATION('',$,#17214);
#17207=APPLICATION_CONTEXT(
'Core Data for Automotive Mechanical Design Process');
#17208=PRODUCT_CONTEXT('part definition',#17207,'mechanical');
#17214=PRODUCT('Guide shaft support','Guide shaft support',
'Guide shaft support',(#17208));
#17320=COLOUR_RGB('Grey',0.48,0.52,0.57);
#17321=FILL_AREA_STYLE_COLOUR('',#17320);
#17322=FILL_AREA_STYLE('',(#17321));
#17323=SURFACE_STYLE_FILL_AREA(#17322);
#17324=SURFACE_SIDE_STYLE('',(#17323));
#17325=SURFACE_STYLE_USAGE(.BOTH.,#17324);
#17326=PRESENTATION_STYLE_ASSIGNMENT((#17325));
ENDSEC;
END-ISO-10303-21;
